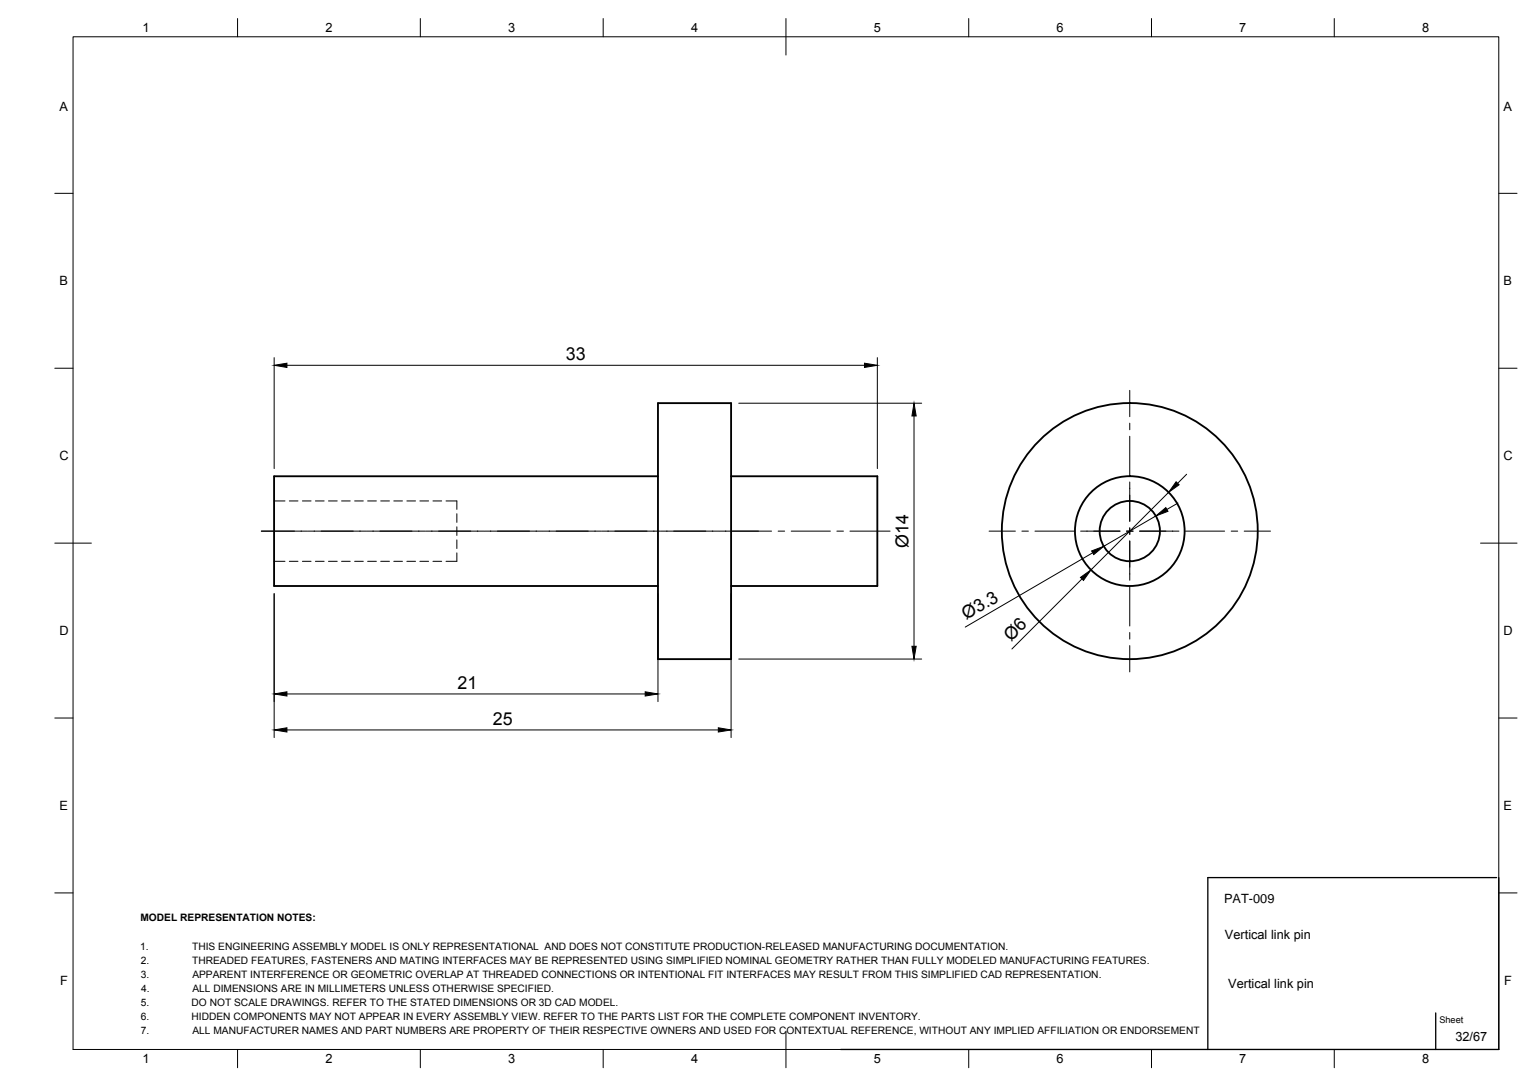
ISO-10303-21;
HEADER;
/* Generated by software containing ST-Developer
 * from STEP Tools, Inc. (www.steptools.com) 
 */

FILE_DESCRIPTION(
/* description */ ('Bell-crank linkage with push rods'),
/* implementation_level */ '2;1');

FILE_NAME(
/* name */ 'Vertical link pin.step',
/* time_stamp */ '2026-10-28T03:25:15-07:00',
/* author */ (''),
/* organization */ (''),
/* preprocessor_version */ 'ST-DEVELOPER v20.2',
/* originating_system */ 'Autodesk Translation Framework v15.17.0.0',
/* authorisation */ '');

FILE_SCHEMA (('AUTOMOTIVE_DESIGN { 1 0 10303 214 3 1 1 }'));
ENDSEC;

DATA;
#10=MECHANICAL_DESIGN_GEOMETRIC_PRESENTATION_REPRESENTATION('',(#637),#16678);
#521=SHAPE_REPRESENTATION_RELATIONSHIP('SRR','None',#16939,#575);
#575=ADVANCED_BREP_SHAPE_REPRESENTATION('',(#698),#16644);
#637=STYLED_ITEM('',(#17291),#698);
#698=MANIFOLD_SOLID_BREP('Body1',#8828);
#847=FACE_BOUND('',#2182,.T.);
#848=FACE_BOUND('',#2184,.T.);
#849=FACE_BOUND('',#2189,.T.);
#1112=PLANE('',#10074);
#1113=PLANE('',#10075);
#1114=PLANE('',#10078);
#1115=PLANE('',#10086);
#1116=PLANE('',#10087);
#1535=FACE_OUTER_BOUND('',#2179,.T.);
#1536=FACE_OUTER_BOUND('',#2180,.T.);
#1537=FACE_OUTER_BOUND('',#2181,.T.);
#1538=FACE_OUTER_BOUND('',#2183,.T.);
#1539=FACE_OUTER_BOUND('',#2185,.T.);
#1540=FACE_OUTER_BOUND('',#2186,.T.);
#1541=FACE_OUTER_BOUND('',#2187,.T.);
#1542=FACE_OUTER_BOUND('',#2188,.T.);
#1543=FACE_OUTER_BOUND('',#2190,.T.);
#2179=EDGE_LOOP('',(#7165,#7166,#7167,#7168));
#2180=EDGE_LOOP('',(#7169));
#2181=EDGE_LOOP('',(#7170));
#2182=EDGE_LOOP('',(#7171));
#2183=EDGE_LOOP('',(#7172));
#2184=EDGE_LOOP('',(#7173));
#2185=EDGE_LOOP('',(#7174,#7175,#7176,#7177));
#2186=EDGE_LOOP('',(#7178,#7179,#7180,#7181));
#2187=EDGE_LOOP('',(#7182,#7183,#7184,#7185));
#2188=EDGE_LOOP('',(#7186));
#2189=EDGE_LOOP('',(#7187));
#2190=EDGE_LOOP('',(#7188));
#2826=LINE('',#15443,#3375);
#2827=LINE('',#15457,#3376);
#2828=LINE('',#15460,#3377);
#2829=LINE('',#15465,#3378);
#3375=VECTOR('',#12162,0.165);
#3376=VECTOR('',#12181,0.7);
#3377=VECTOR('',#12184,0.3);
#3378=VECTOR('',#12191,0.3);
#3924=CIRCLE('',#10072,0.165);
#3925=CIRCLE('',#10073,0.165);
#3926=CIRCLE('',#10076,0.7);
#3927=CIRCLE('',#10077,0.3);
#3928=CIRCLE('',#10079,0.7);
#3929=CIRCLE('',#10080,0.3);
#3930=CIRCLE('',#10083,0.3);
#3931=CIRCLE('',#10085,0.3);
#4535=VERTEX_POINT('',#15440);
#4536=VERTEX_POINT('',#15442);
#4537=VERTEX_POINT('',#15447);
#4538=VERTEX_POINT('',#15449);
#4539=VERTEX_POINT('',#15452);
#4540=VERTEX_POINT('',#15454);
#4541=VERTEX_POINT('',#15459);
#4542=VERTEX_POINT('',#15463);
#5460=EDGE_CURVE('',#4535,#4535,#3924,.T.);
#5461=EDGE_CURVE('',#4535,#4536,#2826,.T.);
#5462=EDGE_CURVE('',#4536,#4536,#3925,.T.);
#5463=EDGE_CURVE('',#4537,#4537,#3926,.T.);
#5464=EDGE_CURVE('',#4538,#4538,#3927,.T.);
#5465=EDGE_CURVE('',#4539,#4539,#3928,.T.);
#5466=EDGE_CURVE('',#4540,#4540,#3929,.T.);
#5467=EDGE_CURVE('',#4537,#4539,#2827,.T.);
#5468=EDGE_CURVE('',#4540,#4541,#2828,.T.);
#5469=EDGE_CURVE('',#4541,#4541,#3930,.T.);
#5470=EDGE_CURVE('',#4542,#4542,#3931,.T.);
#5471=EDGE_CURVE('',#4542,#4538,#2829,.T.);
#7165=ORIENTED_EDGE('',*,*,#5460,.F.);
#7166=ORIENTED_EDGE('',*,*,#5461,.T.);
#7167=ORIENTED_EDGE('',*,*,#5462,.F.);
#7168=ORIENTED_EDGE('',*,*,#5461,.F.);
#7169=ORIENTED_EDGE('',*,*,#5460,.T.);
#7170=ORIENTED_EDGE('',*,*,#5463,.T.);
#7171=ORIENTED_EDGE('',*,*,#5464,.F.);
#7172=ORIENTED_EDGE('',*,*,#5465,.F.);
#7173=ORIENTED_EDGE('',*,*,#5466,.F.);
#7174=ORIENTED_EDGE('',*,*,#5463,.F.);
#7175=ORIENTED_EDGE('',*,*,#5467,.T.);
#7176=ORIENTED_EDGE('',*,*,#5465,.T.);
#7177=ORIENTED_EDGE('',*,*,#5467,.F.);
#7178=ORIENTED_EDGE('',*,*,#5466,.T.);
#7179=ORIENTED_EDGE('',*,*,#5468,.T.);
#7180=ORIENTED_EDGE('',*,*,#5469,.T.);
#7181=ORIENTED_EDGE('',*,*,#5468,.F.);
#7182=ORIENTED_EDGE('',*,*,#5470,.F.);
#7183=ORIENTED_EDGE('',*,*,#5471,.T.);
#7184=ORIENTED_EDGE('',*,*,#5464,.T.);
#7185=ORIENTED_EDGE('',*,*,#5471,.F.);
#7186=ORIENTED_EDGE('',*,*,#5470,.T.);
#7187=ORIENTED_EDGE('',*,*,#5462,.T.);
#7188=ORIENTED_EDGE('',*,*,#5469,.F.);
#8181=CYLINDRICAL_SURFACE('',#10071,0.165);
#8182=CYLINDRICAL_SURFACE('',#10081,0.7);
#8183=CYLINDRICAL_SURFACE('',#10082,0.3);
#8184=CYLINDRICAL_SURFACE('',#10084,0.3);
#8560=ADVANCED_FACE('',(#1535),#8181,.F.);
#8561=ADVANCED_FACE('',(#1536),#1112,.T.);
#8562=ADVANCED_FACE('',(#1537,#847),#1113,.T.);
#8563=ADVANCED_FACE('',(#1538,#848),#1114,.F.);
#8564=ADVANCED_FACE('',(#1539),#8182,.T.);
#8565=ADVANCED_FACE('',(#1540),#8183,.T.);
#8566=ADVANCED_FACE('',(#1541),#8184,.T.);
#8567=ADVANCED_FACE('',(#1542,#849),#1115,.T.);
#8568=ADVANCED_FACE('',(#1543),#1116,.F.);
#8828=CLOSED_SHELL('',(#8560,#8561,#8562,#8563,#8564,#8565,#8566,#8567,
#8568));
#10070=AXIS2_PLACEMENT_3D('',#15438,#12156,#12157);
#10071=AXIS2_PLACEMENT_3D('',#15439,#12158,#12159);
#10072=AXIS2_PLACEMENT_3D('',#15441,#12160,#12161);
#10073=AXIS2_PLACEMENT_3D('',#15444,#12163,#12164);
#10074=AXIS2_PLACEMENT_3D('',#15445,#12165,#12166);
#10075=AXIS2_PLACEMENT_3D('',#15446,#12167,#12168);
#10076=AXIS2_PLACEMENT_3D('',#15448,#12169,#12170);
#10077=AXIS2_PLACEMENT_3D('',#15450,#12171,#12172);
#10078=AXIS2_PLACEMENT_3D('',#15451,#12173,#12174);
#10079=AXIS2_PLACEMENT_3D('',#15453,#12175,#12176);
#10080=AXIS2_PLACEMENT_3D('',#15455,#12177,#12178);
#10081=AXIS2_PLACEMENT_3D('',#15456,#12179,#12180);
#10082=AXIS2_PLACEMENT_3D('',#15458,#12182,#12183);
#10083=AXIS2_PLACEMENT_3D('',#15461,#12185,#12186);
#10084=AXIS2_PLACEMENT_3D('',#15462,#12187,#12188);
#10085=AXIS2_PLACEMENT_3D('',#15464,#12189,#12190);
#10086=AXIS2_PLACEMENT_3D('',#15466,#12192,#12193);
#10087=AXIS2_PLACEMENT_3D('',#15467,#12194,#12195);
#12156=DIRECTION('axis',(0.,0.,1.));
#12157=DIRECTION('refdir',(1.,0.,0.));
#12158=DIRECTION('center_axis',(0.,0.,1.));
#12159=DIRECTION('ref_axis',(1.,0.,0.));
#12160=DIRECTION('center_axis',(0.,0.,1.));
#12161=DIRECTION('ref_axis',(1.,0.,0.));
#12162=DIRECTION('',(0.,0.,1.));
#12163=DIRECTION('center_axis',(0.,0.,-1.));
#12164=DIRECTION('ref_axis',(1.,0.,0.));
#12165=DIRECTION('center_axis',(0.,0.,1.));
#12166=DIRECTION('ref_axis',(1.,0.,0.));
#12167=DIRECTION('center_axis',(0.,0.,1.));
#12168=DIRECTION('ref_axis',(1.,0.,0.));
#12169=DIRECTION('center_axis',(0.,0.,1.));
#12170=DIRECTION('ref_axis',(1.,0.,0.));
#12171=DIRECTION('center_axis',(0.,0.,1.));
#12172=DIRECTION('ref_axis',(1.,0.,0.));
#12173=DIRECTION('center_axis',(0.,0.,1.));
#12174=DIRECTION('ref_axis',(1.,0.,0.));
#12175=DIRECTION('center_axis',(0.,0.,1.));
#12176=DIRECTION('ref_axis',(1.,0.,0.));
#12177=DIRECTION('center_axis',(0.,0.,-1.));
#12178=DIRECTION('ref_axis',(1.,0.,0.));
#12179=DIRECTION('center_axis',(0.,0.,1.));
#12180=DIRECTION('ref_axis',(1.,0.,0.));
#12181=DIRECTION('',(0.,0.,-1.));
#12182=DIRECTION('center_axis',(0.,0.,1.));
#12183=DIRECTION('ref_axis',(1.,0.,0.));
#12184=DIRECTION('',(0.,0.,-1.));
#12185=DIRECTION('center_axis',(0.,0.,1.));
#12186=DIRECTION('ref_axis',(1.,0.,0.));
#12187=DIRECTION('center_axis',(0.,0.,1.));
#12188=DIRECTION('ref_axis',(1.,0.,0.));
#12189=DIRECTION('center_axis',(0.,0.,1.));
#12190=DIRECTION('ref_axis',(1.,0.,0.));
#12191=DIRECTION('',(0.,0.,-1.));
#12192=DIRECTION('center_axis',(0.,0.,1.));
#12193=DIRECTION('ref_axis',(1.,0.,0.));
#12194=DIRECTION('center_axis',(0.,0.,1.));
#12195=DIRECTION('ref_axis',(1.,0.,0.));
#15438=CARTESIAN_POINT('',(0.,0.,0.));
#15439=CARTESIAN_POINT('Origin',(4.,0.,7.1));
#15440=CARTESIAN_POINT('',(3.835,-2.02066721859313E-17,7.1));
#15441=CARTESIAN_POINT('Origin',(4.,0.,7.1));
#15442=CARTESIAN_POINT('',(3.835,2.02066721859313E-17,8.1));
#15443=CARTESIAN_POINT('',(3.835,-2.02066721859313E-17,7.1));
#15444=CARTESIAN_POINT('Origin',(4.,0.,8.1));
#15445=CARTESIAN_POINT('Origin',(4.,0.,7.1));
#15446=CARTESIAN_POINT('Origin',(4.,0.,6.));
#15447=CARTESIAN_POINT('',(3.3,-8.57252759403147E-17,6.));
#15448=CARTESIAN_POINT('Origin',(4.,0.,6.));
#15449=CARTESIAN_POINT('',(3.7,-3.67394039744206E-17,6.));
#15450=CARTESIAN_POINT('Origin',(4.,0.,6.));
#15451=CARTESIAN_POINT('Origin',(4.,0.,5.6));
#15452=CARTESIAN_POINT('',(3.3,-8.57252759403147E-17,5.6));
#15453=CARTESIAN_POINT('Origin',(4.,0.,5.6));
#15454=CARTESIAN_POINT('',(3.7,3.67394039744206E-17,5.6));
#15455=CARTESIAN_POINT('Origin',(4.,0.,5.6));
#15456=CARTESIAN_POINT('Origin',(4.,0.,5.6));
#15457=CARTESIAN_POINT('',(3.3,-8.57252759403147E-17,5.6));
#15458=CARTESIAN_POINT('Origin',(4.,0.,4.8));
#15459=CARTESIAN_POINT('',(3.7,-3.67394039744206E-17,4.8));
#15460=CARTESIAN_POINT('',(3.7,-3.67394039744206E-17,4.8));
#15461=CARTESIAN_POINT('Origin',(4.,0.,4.8));
#15462=CARTESIAN_POINT('Origin',(4.,0.,4.8));
#15463=CARTESIAN_POINT('',(3.7,-3.67394039744206E-17,8.1));
#15464=CARTESIAN_POINT('Origin',(4.,0.,8.1));
#15465=CARTESIAN_POINT('',(3.7,-3.67394039744206E-17,4.8));
#15466=CARTESIAN_POINT('Origin',(4.,0.,8.1));
#15467=CARTESIAN_POINT('Origin',(4.,0.,4.8));
#16580=UNCERTAINTY_MEASURE_WITH_UNIT(LENGTH_MEASURE(0.001),#16679,
'DISTANCE_ACCURACY_VALUE',
'Maximum model space distance between geometric entities at asserted c
onnectivities');
#16614=UNCERTAINTY_MEASURE_WITH_UNIT(LENGTH_MEASURE(0.001),#16679,
'DISTANCE_ACCURACY_VALUE',
'Maximum model space distance between geometric entities at asserted c
onnectivities');
#16644=(
GEOMETRIC_REPRESENTATION_CONTEXT(3)
GLOBAL_UNCERTAINTY_ASSIGNED_CONTEXT((#16580))
GLOBAL_UNIT_ASSIGNED_CONTEXT((#16679,#16681,#16682))
REPRESENTATION_CONTEXT('','3D')
);
#16678=(
GEOMETRIC_REPRESENTATION_CONTEXT(3)
GLOBAL_UNCERTAINTY_ASSIGNED_CONTEXT((#16614))
GLOBAL_UNIT_ASSIGNED_CONTEXT((#16679,#16681,#16682))
REPRESENTATION_CONTEXT('','3D')
);
#16679=(
LENGTH_UNIT()
NAMED_UNIT(*)
SI_UNIT(.CENTI.,.METRE.)
);
#16681=(
NAMED_UNIT(*)
PLANE_ANGLE_UNIT()
SI_UNIT($,.RADIAN.)
);
#16682=(
NAMED_UNIT(*)
SI_UNIT($,.STERADIAN.)
SOLID_ANGLE_UNIT()
);
#16712=SHAPE_DEFINITION_REPRESENTATION(#16780,#16939);
#16780=PRODUCT_DEFINITION_SHAPE('',$,#17003);
#16939=SHAPE_REPRESENTATION('',(#10070),#16644);
#16973=PRODUCT_DEFINITION_CONTEXT('part definition',#17164,'design');
#17003=PRODUCT_DEFINITION('Vertical link pin','Vertical link pin',#17066,
#16973);
#17066=PRODUCT_DEFINITION_FORMATION('',$,#17195);
#17164=APPLICATION_CONTEXT(
'Core Data for Automotive Mechanical Design Process');
#17165=PRODUCT_CONTEXT('part definition',#17164,'mechanical');
#17195=PRODUCT('Vertical link pin','Vertical link pin',
'Vertical link pin',(#17165));
#17285=COLOUR_RGB('Grey',0.48,0.52,0.57);
#17286=FILL_AREA_STYLE_COLOUR('',#17285);
#17287=FILL_AREA_STYLE('',(#17286));
#17288=SURFACE_STYLE_FILL_AREA(#17287);
#17289=SURFACE_SIDE_STYLE('',(#17288));
#17290=SURFACE_STYLE_USAGE(.BOTH.,#17289);
#17291=PRESENTATION_STYLE_ASSIGNMENT((#17290));
ENDSEC;
END-ISO-10303-21;
